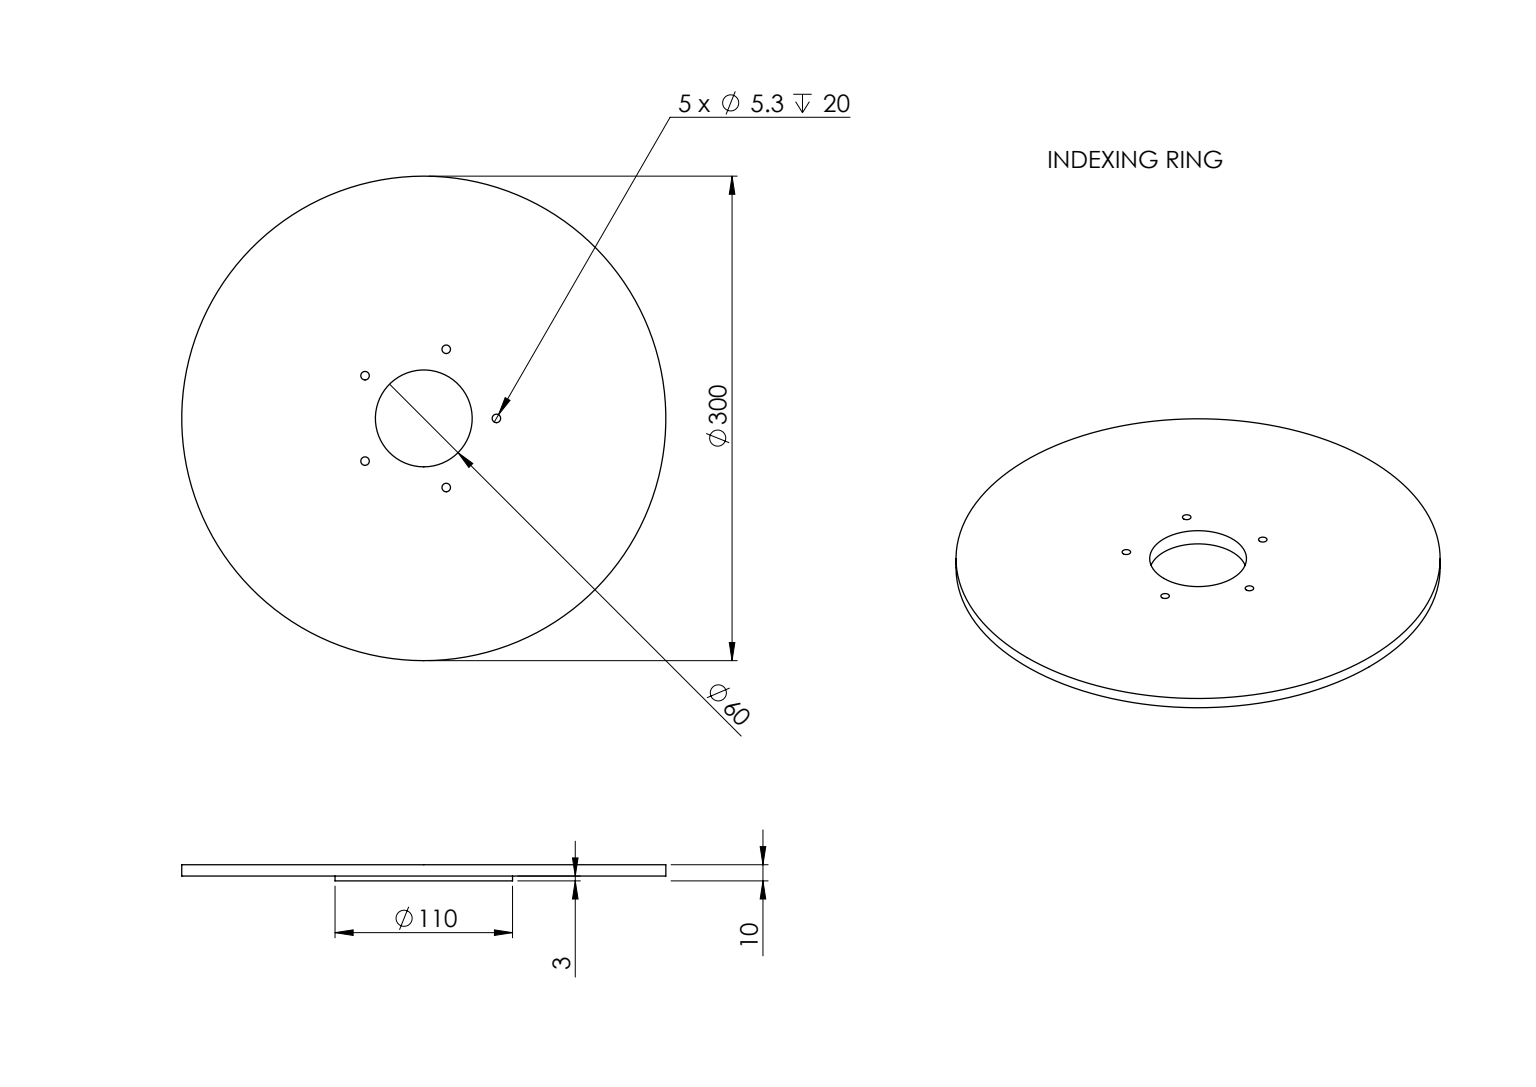
ISO-10303-21;
HEADER;
FILE_DESCRIPTION (('STEP AP214'),
    '1' );
FILE_NAME ('Indexing Ring.step',
    '2026-10-24T07:08:27',
    ( '' ),
    ( '' ),
    'SwSTEP 2.0',
    'SolidWorks 2026',
    '' );
FILE_SCHEMA (( 'AUTOMOTIVE_DESIGN' ));
ENDSEC;

DATA;
#5=CIRCLE ( 'NONE', #16107, 2.649999999999999467 ) ;
#16=ORIENTED_EDGE ( 'NONE', *, *, #15782, .F. ) ;
#43=AXIS2_PLACEMENT_3D ( 'NONE', #4578, #2974, #8946 ) ;
#70=DIRECTION ( 'NONE',  ( 0.000000000000000000, 0.000000000000000000, 1.000000000000000000 ) ) ;
#74=VECTOR ( 'NONE', #5888, 1000.000000000000000 ) ;
#109=DIRECTION ( 'NONE',  ( -0.000000000000000000, 1.000000000000000000, -0.000000000000000000 ) ) ;
#135=CARTESIAN_POINT ( 'NONE',  ( 13.90576474687299680, 0.000000000000000000, 42.79754323328179311 ) ) ;
#142=LINE ( 'NONE', #1937, #2927 ) ;
#166=CYLINDRICAL_SURFACE ( 'NONE', #15609, 30.00000000000000000 ) ;
#204=CYLINDRICAL_SURFACE ( 'NONE', #43, 55.00000000000000000 ) ;
#220=EDGE_CURVE ( 'NONE', #7351, #4921, #14999, .T. ) ;
#273=ORIENTED_EDGE ( 'NONE', *, *, #14374, .F. ) ;
#286=DIRECTION ( 'NONE',  ( -0.000000000000000000, -1.000000000000000000, -0.000000000000000000 ) ) ;
#301=ORIENTED_EDGE ( 'NONE', *, *, #12426, .F. ) ;
#305=EDGE_CURVE ( 'NONE', #13142, #9008, #11661, .T. ) ;
#340=ORIENTED_EDGE ( 'NONE', *, *, #305, .F. ) ;
#390=DIRECTION ( 'NONE',  ( 0.000000000000000000, -1.000000000000000000, 0.000000000000000000 ) ) ;
#402=EDGE_CURVE ( 'NONE', #11928, #9088, #2271, .T. ) ;
#413=CARTESIAN_POINT ( 'NONE',  ( 0.000000000000000000, 3.000000000000000000, 0.000000000000000000 ) ) ;
#469=DIRECTION ( 'NONE',  ( -0.000000000000000000, 1.000000000000000000, -0.000000000000000000 ) ) ;
#486=( LENGTH_UNIT ( ) NAMED_UNIT ( * ) SI_UNIT ( .MILLI., .METRE. ) );
#520=ORIENTED_EDGE ( 'NONE', *, *, #14011, .T. ) ;
#640=ORIENTED_EDGE ( 'NONE', *, *, #15047, .T. ) ;
#641=EDGE_CURVE ( 'NONE', #14362, #16890, #13288, .T. ) ;
#689=AXIS2_PLACEMENT_3D ( 'NONE', #18645, #7031, #2265 ) ;
#779=AXIS2_PLACEMENT_3D ( 'NONE', #6879, #12893, #15840 ) ;
#880=EDGE_CURVE ( 'NONE', #14362, #3677, #9321, .T. ) ;
#898=CARTESIAN_POINT ( 'NONE',  ( 13.90576474687263264, 0.000000000000000000, -42.79754323328189969 ) ) ;
#940=DIRECTION ( 'NONE',  ( 0.000000000000000000, 0.000000000000000000, 1.000000000000000000 ) ) ;
#955=ORIENTED_EDGE ( 'NONE', *, *, #4704, .T. ) ;
#967=CARTESIAN_POINT ( 'NONE',  ( 13.90576474687263264, 0.000000000000000000, -40.14754323328190111 ) ) ;
#970=ORIENTED_EDGE ( 'NONE', *, *, #12368, .T. ) ;
#982=CARTESIAN_POINT ( 'NONE',  ( 0.000000000000000000, 10.00000000000000000, -30.00000000000000000 ) ) ;
#991=DIRECTION ( 'NONE',  ( 0.000000000000000000, 0.000000000000000000, 1.000000000000000000 ) ) ;
#1029=EDGE_LOOP ( 'NONE', ( #970, #3446 ) ) ;
#1070=CARTESIAN_POINT ( 'NONE',  ( -36.40576474687271258, 10.00000000000000000, -26.45033635316118747 ) ) ;
#1105=AXIS2_PLACEMENT_3D ( 'NONE', #4053, #17378, #12810 ) ;
#1236=CYLINDRICAL_SURFACE ( 'NONE', #689, 2.649999999999999467 ) ;
#1286=AXIS2_PLACEMENT_3D ( 'NONE', #17811, #8951, #10577 ) ;
#1294=DIRECTION ( 'NONE',  ( 0.000000000000000000, 0.000000000000000000, 1.000000000000000000 ) ) ;
#1343=EDGE_LOOP ( 'NONE', ( #520, #9190 ) ) ;
#1397=EDGE_LOOP ( 'NONE', ( #11377, #14520, #10547, #14301 ) ) ;
#1452=CIRCLE ( 'NONE', #12089, 2.649999999999999467 ) ;
#1510=ADVANCED_FACE ( 'NONE', ( #15262, #2212 ), #17837, .T. ) ;
#1524=LINE ( 'NONE', #13055, #14054 ) ;
#1532=DIRECTION ( 'NONE',  ( 0.000000000000000000, -1.000000000000000000, 0.000000000000000000 ) ) ;
#1540=ORIENTED_EDGE ( 'NONE', *, *, #641, .F. ) ;
#1585=ORIENTED_EDGE ( 'NONE', *, *, #17375, .F. ) ;
#1675=AXIS2_PLACEMENT_3D ( 'NONE', #9927, #15556, #991 ) ;
#1709=AXIS2_PLACEMENT_3D ( 'NONE', #3286, #16430, #8983 ) ;
#1710=ADVANCED_FACE ( 'NONE', ( #9924 ), #17174, .F. ) ;
#1765=CARTESIAN_POINT ( 'NONE',  ( 0.000000000000000000, 3.000000000000000000, 0.000000000000000000 ) ) ;
#1859=DIRECTION ( 'NONE',  ( -0.000000000000000000, -1.000000000000000000, -0.000000000000000000 ) ) ;
#1868=LINE ( 'NONE', #16163, #9313 ) ;
#1911=DIRECTION ( 'NONE',  ( 1.000000000000000000, 0.000000000000000000, 0.000000000000000000 ) ) ;
#1926=ORIENTED_EDGE ( 'NONE', *, *, #12328, .F. ) ;
#1937=CARTESIAN_POINT ( 'NONE',  ( -36.40576474687271258, 10.00000000000000000, -29.10033635316118961 ) ) ;
#1938=LINE ( 'NONE', #6417, #10148 ) ;
#1963=CARTESIAN_POINT ( 'NONE',  ( -36.40576474687271258, 10.00000000000000000, -29.10033635316118961 ) ) ;
#1966=DIRECTION ( 'NONE',  ( -0.000000000000000000, 1.000000000000000000, -0.000000000000000000 ) ) ;
#1971=AXIS2_PLACEMENT_3D ( 'NONE', #11706, #4557, #7409 ) ;
#1981=CARTESIAN_POINT ( 'NONE',  ( 45.00000000000000000, 10.00000000000000000, -2.650000000000511946 ) ) ;
#1996=EDGE_LOOP ( 'NONE', ( #7930, #18641, #8266, #16907 ) ) ;
#2097=AXIS2_PLACEMENT_3D ( 'NONE', #16593, #15458, #3830 ) ;
#2107=VERTEX_POINT ( 'NONE', #967 ) ;
#2121=CYLINDRICAL_SURFACE ( 'NONE', #16679, 150.0000000000000284 ) ;
#2123=DIRECTION ( 'NONE',  ( 0.000000000000000000, -1.000000000000000000, 0.000000000000000000 ) ) ;
#2158=ORIENTED_EDGE ( 'NONE', *, *, #18549, .T. ) ;
#2212=FACE_OUTER_BOUND ( 'NONE', #3227, .T. ) ;
#2223=CLOSED_SHELL ( 'NONE', ( #15200, #17927, #1710, #5636, #4878, #2825, #17976, #16218, #14114, #15768, #13678, #3090, #12859, #4334, #4412, #8329, #14903, #1510, #9932 ) ) ;
#2253=CYLINDRICAL_SURFACE ( 'NONE', #7817, 2.649999999999999467 ) ;
#2265=DIRECTION ( 'NONE',  ( 0.000000000000000000, 0.000000000000000000, 1.000000000000000000 ) ) ;
#2271=LINE ( 'NONE', #15705, #10103 ) ;
#2500=DIRECTION ( 'NONE',  ( 0.000000000000000000, -1.000000000000000000, 0.000000000000000000 ) ) ;
#2501=DIRECTION ( 'NONE',  ( -0.000000000000000000, 1.000000000000000000, -0.000000000000000000 ) ) ;
#2534=DIRECTION ( 'NONE',  ( -0.000000000000000000, 1.000000000000000000, -0.000000000000000000 ) ) ;
#2568=DIRECTION ( 'NONE',  ( -0.000000000000000000, 1.000000000000000000, -0.000000000000000000 ) ) ;
#2580=EDGE_LOOP ( 'NONE', ( #4963, #18151 ) ) ;
#2605=ORIENTED_EDGE ( 'NONE', *, *, #12034, .T. ) ;
#2612=CIRCLE ( 'NONE', #6253, 2.649999999999999467 ) ;
#2736=FACE_BOUND ( 'NONE', #8126, .T. ) ;
#2771=ORIENTED_EDGE ( 'NONE', *, *, #13030, .F. ) ;
#2778=ORIENTED_EDGE ( 'NONE', *, *, #402, .T. ) ;
#2794=SURFACE_STYLE_USAGE ( .BOTH. , #11462 ) ;
#2801=CIRCLE ( 'NONE', #12208, 150.0000000000000000 ) ;
#2803=PLANE ( 'NONE',  #1105 ) ;
#2804=CARTESIAN_POINT ( 'NONE',  ( 45.00000000000000000, 10.00000000000000000, 2.649999999999487432 ) ) ;
#2825=ADVANCED_FACE ( 'NONE', ( #5792 ), #4360, .F. ) ;
#2829=ORIENTED_EDGE ( 'NONE', *, *, #16831, .T. ) ;
#2845=AXIS2_PLACEMENT_3D ( 'NONE', #15238, #14861, #10564 ) ;
#2891=EDGE_CURVE ( 'NONE', #3956, #15653, #1868, .T. ) ;
#2903=CARTESIAN_POINT ( 'NONE',  ( 6.735557395310442615E-15, 0.000000000000000000, 55.00000000000000000 ) ) ;
#2913=AXIS2_PLACEMENT_3D ( 'NONE', #6516, #7946, #6621 ) ;
#2927=VECTOR ( 'NONE', #13281, 1000.000000000000000 ) ;
#2974=DIRECTION ( 'NONE',  ( -0.000000000000000000, -1.000000000000000000, -0.000000000000000000 ) ) ;
#3025=ORIENTED_EDGE ( 'NONE', *, *, #8650, .T. ) ;
#3090=ADVANCED_FACE ( 'NONE', ( #5286 ), #12440, .F. ) ;
#3120=EDGE_CURVE ( 'NONE', #18403, #16590, #6572, .T. ) ;
#3227=EDGE_LOOP ( 'NONE', ( #14533, #10465 ) ) ;
#3286=CARTESIAN_POINT ( 'NONE',  ( -36.40576474687247099, 10.00000000000000000, 26.45033635316149301 ) ) ;
#3310=EDGE_CURVE ( 'NONE', #6304, #3994, #142, .T. ) ;
#3354=CARTESIAN_POINT ( 'NONE',  ( 45.00000000000000000, 0.000000000000000000, 2.649999999999487432 ) ) ;
#3396=CIRCLE ( 'NONE', #1286, 2.649999999999999467 ) ;
#3446=ORIENTED_EDGE ( 'NONE', *, *, #12426, .T. ) ;
#3501=CIRCLE ( 'NONE', #4120, 55.00000000000000000 ) ;
#3517=VERTEX_POINT ( 'NONE', #15824 ) ;
#3585=DIRECTION ( 'NONE',  ( 0.000000000000000000, 0.000000000000000000, -1.000000000000000000 ) ) ;
#3631=ORIENTED_EDGE ( 'NONE', *, *, #12034, .F. ) ;
#3632=CARTESIAN_POINT ( 'NONE',  ( 0.000000000000000000, 0.000000000000000000, 0.000000000000000000 ) ) ;
#3677=VERTEX_POINT ( 'NONE', #6089 ) ;
#3705=EDGE_LOOP ( 'NONE', ( #16152, #4220 ) ) ;
#3735=VECTOR ( 'NONE', #12593, 1000.000000000000000 ) ;
#3737=ORIENTED_EDGE ( 'NONE', *, *, #17718, .F. ) ;
#3785=EDGE_LOOP ( 'NONE', ( #10703, #14581, #9081, #11061 ) ) ;
#3830=DIRECTION ( 'NONE',  ( 0.000000000000000000, 0.000000000000000000, -1.000000000000000000 ) ) ;
#3940=DIRECTION ( 'NONE',  ( 0.000000000000000000, 1.000000000000000000, 0.000000000000000000 ) ) ;
#3956=VERTEX_POINT ( 'NONE', #7399 ) ;
#3994=VERTEX_POINT ( 'NONE', #1963 ) ;
#4039=DIRECTION ( 'NONE',  ( 0.000000000000000000, 0.000000000000000000, 1.000000000000000000 ) ) ;
#4045=CARTESIAN_POINT ( 'NONE',  ( 45.00000000000000000, 0.000000000000000000, -5.120903701083534543E-13 ) ) ;
#4053=CARTESIAN_POINT ( 'NONE',  ( 0.000000000000000000, 0.000000000000000000, 0.000000000000000000 ) ) ;
#4120=AXIS2_PLACEMENT_3D ( 'NONE', #18310, #11060, #16887 ) ;
#4185=EDGE_CURVE ( 'NONE', #9008, #13142, #2612, .T. ) ;
#4198=CARTESIAN_POINT ( 'NONE',  ( -36.40576474687247099, 10.00000000000000000, 29.10033635316149514 ) ) ;
#4206=FACE_OUTER_BOUND ( 'NONE', #12915, .T. ) ;
#4220=ORIENTED_EDGE ( 'NONE', *, *, #17207, .T. ) ;
#4246=DIRECTION ( 'NONE',  ( 0.000000000000000000, 1.000000000000000000, 0.000000000000000000 ) ) ;
#4296=ORIENTED_EDGE ( 'NONE', *, *, #9114, .T. ) ;
#4313=CIRCLE ( 'NONE', #6737, 150.0000000000000284 ) ;
#4334=ADVANCED_FACE ( 'NONE', ( #10146 ), #17204, .F. ) ;
#4355=FACE_OUTER_BOUND ( 'NONE', #10583, .T. ) ;
#4360=CYLINDRICAL_SURFACE ( 'NONE', #12135, 2.649999999999999467 ) ;
#4363=VERTEX_POINT ( 'NONE', #5495 ) ;
#4412=ADVANCED_FACE ( 'NONE', ( #13572 ), #7653, .F. ) ;
#4424=VECTOR ( 'NONE', #9470, 1000.000000000000000 ) ;
#4439=DIRECTION ( 'NONE',  ( -0.000000000000000000, 1.000000000000000000, -0.000000000000000000 ) ) ;
#4464=FACE_OUTER_BOUND ( 'NONE', #5126, .T. ) ;
#4465=AXIS2_PLACEMENT_3D ( 'NONE', #5371, #9941, #15755 ) ;
#4479=CARTESIAN_POINT ( 'NONE',  ( -36.40576474687271258, 10.00000000000000000, -26.45033635316118747 ) ) ;
#4491=( LENGTH_UNIT ( ) NAMED_UNIT ( * ) SI_UNIT ( .MILLI., .METRE. ) );
#4504=( NAMED_UNIT ( * ) PLANE_ANGLE_UNIT ( ) SI_UNIT ( $, .RADIAN. ) );
#4530=ORIENTED_EDGE ( 'NONE', *, *, #17601, .F. ) ;
#4557=DIRECTION ( 'NONE',  ( -0.000000000000000000, -1.000000000000000000, -0.000000000000000000 ) ) ;
#4578=CARTESIAN_POINT ( 'NONE',  ( 0.000000000000000000, 3.000000000000000000, 0.000000000000000000 ) ) ;
#4581=( NAMED_UNIT ( * ) PLANE_ANGLE_UNIT ( ) SI_UNIT ( $, .RADIAN. ) );
#4630=APPLICATION_CONTEXT ( 'automotive_design' ) ;
#4662=CYLINDRICAL_SURFACE ( 'NONE', #14552, 2.649999999999999467 ) ;
#4673=PRODUCT_DEFINITION ( 'UNKNOWN', '', #8673, #14538 ) ;
#4704=EDGE_CURVE ( 'NONE', #16890, #11456, #12037, .T. ) ;
#4754=FACE_OUTER_BOUND ( 'NONE', #5207, .T. ) ;
#4769=AXIS2_PLACEMENT_3D ( 'NONE', #17245, #16087, #10275 ) ;
#4796=DIRECTION ( 'NONE',  ( -0.000000000000000000, 1.000000000000000000, -0.000000000000000000 ) ) ;
#4878=ADVANCED_FACE ( 'NONE', ( #4464 ), #9998, .F. ) ;
#4911=EDGE_CURVE ( 'NONE', #16590, #14829, #7043, .T. ) ;
#4921=VERTEX_POINT ( 'NONE', #18756 ) ;
#4963=ORIENTED_EDGE ( 'NONE', *, *, #9468, .T. ) ;
#4969=COLOUR_RGB ( '',0.8941176470588234615, 0.8941176470588234615, 0.8941176470588234615 ) ;
#5121=ORIENTED_EDGE ( 'NONE', *, *, #17375, .T. ) ;
#5126=EDGE_LOOP ( 'NONE', ( #10625, #10506, #16849, #1585 ) ) ;
#5157=EDGE_CURVE ( 'NONE', #9088, #10404, #9039, .T. ) ;
#5177=ORIENTED_EDGE ( 'NONE', *, *, #17207, .F. ) ;
#5195=DIRECTION ( 'NONE',  ( -0.000000000000000000, -1.000000000000000000, -0.000000000000000000 ) ) ;
#5201=DIRECTION ( 'NONE',  ( -0.000000000000000000, 1.000000000000000000, -0.000000000000000000 ) ) ;
#5207=EDGE_LOOP ( 'NONE', ( #10879, #7424, #17278, #10605 ) ) ;
#5276=CARTESIAN_POINT ( 'NONE',  ( 13.90576474687299680, 10.00000000000000000, 40.14754323328178742 ) ) ;
#5286=FACE_OUTER_BOUND ( 'NONE', #18515, .T. ) ;
#5365=CIRCLE ( 'NONE', #16947, 2.649999999999999467 ) ;
#5371=CARTESIAN_POINT ( 'NONE',  ( 0.000000000000000000, 10.00000000000000000, 0.000000000000000000 ) ) ;
#5393=DIRECTION ( 'NONE',  ( 0.000000000000000000, 0.000000000000000000, 1.000000000000000000 ) ) ;
#5472=AXIS2_PLACEMENT_3D ( 'NONE', #13696, #1966, #18155 ) ;
#5485=DIRECTION ( 'NONE',  ( 0.000000000000000000, -1.000000000000000000, 0.000000000000000000 ) ) ;
#5494=ORIENTED_EDGE ( 'NONE', *, *, #7706, .T. ) ;
#5495=CARTESIAN_POINT ( 'NONE',  ( 45.00000000000000000, 0.000000000000000000, -2.650000000000511946 ) ) ;
#5555=CARTESIAN_POINT ( 'NONE',  ( -36.40576474687271258, 10.00000000000000000, -26.45033635316118747 ) ) ;
#5563=DIRECTION ( 'NONE',  ( 0.000000000000000000, 0.000000000000000000, 1.000000000000000000 ) ) ;
#5578=DIRECTION ( 'NONE',  ( 0.000000000000000000, 1.000000000000000000, 0.000000000000000000 ) ) ;
#5593=EDGE_LOOP ( 'NONE', ( #5669, #6351, #10190, #1540 ) ) ;
#5636=ADVANCED_FACE ( 'NONE', ( #4355 ), #8821, .F. ) ;
#5649=SURFACE_STYLE_FILL_AREA ( #15844 ) ;
#5650=DIRECTION ( 'NONE',  ( 0.000000000000000000, 0.000000000000000000, 1.000000000000000000 ) ) ;
#5659=FACE_BOUND ( 'NONE', #2580, .T. ) ;
#5668=VECTOR ( 'NONE', #286, 1000.000000000000000 ) ;
#5669=ORIENTED_EDGE ( 'NONE', *, *, #880, .T. ) ;
#5682=AXIS2_PLACEMENT_3D ( 'NONE', #1070, #15736, #8401 ) ;
#5700=ORIENTED_EDGE ( 'NONE', *, *, #8890, .F. ) ;
#5706=EDGE_LOOP ( 'NONE', ( #8634, #340 ) ) ;
#5712=ORIENTED_EDGE ( 'NONE', *, *, #3120, .F. ) ;
#5786=EDGE_LOOP ( 'NONE', ( #9980, #17221 ) ) ;
#5792=FACE_OUTER_BOUND ( 'NONE', #18175, .T. ) ;
#5804=FACE_OUTER_BOUND ( 'NONE', #17196, .T. ) ;
#5850=CARTESIAN_POINT ( 'NONE',  ( -36.40576474687247099, 0.000000000000000000, 23.80033635316149443 ) ) ;
#5888=DIRECTION ( 'NONE',  ( -0.000000000000000000, 1.000000000000000000, -0.000000000000000000 ) ) ;
#5929=DIRECTION ( 'NONE',  ( 0.000000000000000000, 1.000000000000000000, 0.000000000000000000 ) ) ;
#5946=LINE ( 'NONE', #8449, #15377 ) ;
#6047=DIRECTION ( 'NONE',  ( -0.000000000000000000, -1.000000000000000000, -0.000000000000000000 ) ) ;
#6089=CARTESIAN_POINT ( 'NONE',  ( 3.673940397442059178E-15, 10.00000000000000000, 30.00000000000000000 ) ) ;
#6119=EDGE_CURVE ( 'NONE', #18371, #8784, #14558, .T. ) ;
#6123=CARTESIAN_POINT ( 'NONE',  ( -36.40576474687271258, 10.00000000000000000, -23.80033635316118890 ) ) ;
#6236=CARTESIAN_POINT ( 'NONE',  ( 6.735557395310442615E-15, 3.000000000000000000, 55.00000000000000000 ) ) ;
#6253=AXIS2_PLACEMENT_3D ( 'NONE', #9396, #5201, #5393 ) ;
#6254=CIRCLE ( 'NONE', #18107, 2.649999999999999467 ) ;
#6261=CARTESIAN_POINT ( 'NONE',  ( 0.000000000000000000, 3.000000000000000000, 0.000000000000000000 ) ) ;
#6304=VERTEX_POINT ( 'NONE', #15354 ) ;
#6337=PRODUCT ( 'Indexing Ring', 'Indexing Ring', '', ( #10128 ) ) ;
#6351=ORIENTED_EDGE ( 'NONE', *, *, #17601, .T. ) ;
#6361=STYLED_ITEM('',(#18890),#15935);
#6375=DIRECTION ( 'NONE',  ( 0.000000000000000000, 0.000000000000000000, 1.000000000000000000 ) ) ;
#6396=( NAMED_UNIT ( * ) SI_UNIT ( $, .STERADIAN. ) SOLID_ANGLE_UNIT ( ) );
#6417=CARTESIAN_POINT ( 'NONE',  ( 13.90576474687263264, 10.00000000000000000, -45.44754323328189827 ) ) ;
#6516=CARTESIAN_POINT ( 'NONE',  ( 0.000000000000000000, 10.00000000000000000, 0.000000000000000000 ) ) ;
#6540=CIRCLE ( 'NONE', #779, 2.649999999999999467 ) ;
#6572=CIRCLE ( 'NONE', #8994, 2.649999999999999467 ) ;
#6618=VECTOR ( 'NONE', #14346, 1000.000000000000000 ) ;
#6621=DIRECTION ( 'NONE',  ( 0.000000000000000000, 0.000000000000000000, 1.000000000000000000 ) ) ;
#6630=AXIS2_PLACEMENT_3D ( 'NONE', #7074, #10212, #5563 ) ;
#6668=MECHANICAL_DESIGN_GEOMETRIC_PRESENTATION_REPRESENTATION('',(#6361),#15787);
#6701=CARTESIAN_POINT ( 'NONE',  ( 0.000000000000000000, 0.000000000000000000, -30.00000000000000000 ) ) ;
#6713=ORIENTED_EDGE ( 'NONE', *, *, #220, .F. ) ;
#6719=CARTESIAN_POINT ( 'NONE',  ( 0.000000000000000000, 0.000000000000000000, 0.000000000000000000 ) ) ;
#6724=DIRECTION ( 'NONE',  ( 0.000000000000000000, 0.000000000000000000, -1.000000000000000000 ) ) ;
#6737=AXIS2_PLACEMENT_3D ( 'NONE', #17449, #8504, #12100 ) ;
#6755=AXIS2_PLACEMENT_3D ( 'NONE', #11426, #11336, #17154 ) ;
#6777=AXIS2_PLACEMENT_3D ( 'NONE', #14577, #1532, #7334 ) ;
#6822=CARTESIAN_POINT ( 'NONE',  ( 13.90576474687263264, 10.00000000000000000, -42.79754323328189969 ) ) ;
#6833=ORIENTED_EDGE ( 'NONE', *, *, #3120, .T. ) ;
#6849=DIRECTION ( 'NONE',  ( 0.000000000000000000, 0.000000000000000000, 1.000000000000000000 ) ) ;
#6856=CARTESIAN_POINT ( 'NONE',  ( 45.00000000000000000, 10.00000000000000000, -5.120903701083534543E-13 ) ) ;
#6879=CARTESIAN_POINT ( 'NONE',  ( -36.40576474687271258, 0.000000000000000000, -26.45033635316118747 ) ) ;
#6976=ORIENTED_EDGE ( 'NONE', *, *, #7706, .F. ) ;
#7000=FACE_BOUND ( 'NONE', #11546, .T. ) ;
#7031=DIRECTION ( 'NONE',  ( -0.000000000000000000, 1.000000000000000000, -0.000000000000000000 ) ) ;
#7043=LINE ( 'NONE', #4198, #17854 ) ;
#7047=CIRCLE ( 'NONE', #17651, 2.649999999999999467 ) ;
#7059=ORIENTED_EDGE ( 'NONE', *, *, #14529, .F. ) ;
#7061=CIRCLE ( 'NONE', #6755, 2.649999999999999467 ) ;
#7074=CARTESIAN_POINT ( 'NONE',  ( -36.40576474687247099, 10.00000000000000000, 26.45033635316149301 ) ) ;
#7107=CARTESIAN_POINT ( 'NONE',  ( 0.000000000000000000, 3.000000000000000000, -55.00000000000000000 ) ) ;
#7198=CARTESIAN_POINT ( 'NONE',  ( 13.90576474687263264, 10.00000000000000000, -40.14754323328190111 ) ) ;
#7208=DIRECTION ( 'NONE',  ( 0.000000000000000000, 0.000000000000000000, -1.000000000000000000 ) ) ;
#7315=CARTESIAN_POINT ( 'NONE',  ( 13.90576474687299680, 0.000000000000000000, 45.44754323328179169 ) ) ;
#7317=CARTESIAN_POINT ( 'NONE',  ( 13.90576474687299680, 10.00000000000000000, 45.44754323328179169 ) ) ;
#7322=DIRECTION ( 'NONE',  ( 1.000000000000000000, 0.000000000000000000, 0.000000000000000000 ) ) ;
#7334=DIRECTION ( 'NONE',  ( 0.000000000000000000, 0.000000000000000000, -1.000000000000000000 ) ) ;
#7351=VERTEX_POINT ( 'NONE', #2903 ) ;
#7399=CARTESIAN_POINT ( 'NONE',  ( -36.40576474687271258, 0.000000000000000000, -23.80033635316118890 ) ) ;
#7409=DIRECTION ( 'NONE',  ( 0.000000000000000000, 0.000000000000000000, -1.000000000000000000 ) ) ;
#7424=ORIENTED_EDGE ( 'NONE', *, *, #12368, .F. ) ;
#7426=FACE_OUTER_BOUND ( 'NONE', #14178, .T. ) ;
#7519=DIRECTION ( 'NONE',  ( 0.000000000000000000, 0.000000000000000000, 1.000000000000000000 ) ) ;
#7562=AXIS2_PLACEMENT_3D ( 'NONE', #13153, #109, #7519 ) ;
#7627=CARTESIAN_POINT ( 'NONE',  ( 13.90576474687263264, 10.00000000000000000, -45.44754323328189827 ) ) ;
#7653=CYLINDRICAL_SURFACE ( 'NONE', #1709, 2.649999999999999467 ) ;
#7706=EDGE_CURVE ( 'NONE', #14393, #14829, #15759, .T. ) ;
#7713=VERTEX_POINT ( 'NONE', #18605 ) ;
#7718=EDGE_CURVE ( 'NONE', #17227, #4363, #1452, .T. ) ;
#7734=EDGE_LOOP ( 'NONE', ( #11489, #16 ) ) ;
#7817=AXIS2_PLACEMENT_3D ( 'NONE', #6822, #8062, #940 ) ;
#7930=ORIENTED_EDGE ( 'NONE', *, *, #18573, .F. ) ;
#7946=DIRECTION ( 'NONE',  ( 0.000000000000000000, 1.000000000000000000, 0.000000000000000000 ) ) ;
#8017=AXIS2_PLACEMENT_3D ( 'NONE', #12801, #14324, #9934 ) ;
#8062=DIRECTION ( 'NONE',  ( -0.000000000000000000, 1.000000000000000000, -0.000000000000000000 ) ) ;
#8100=CARTESIAN_POINT ( 'NONE',  ( 3.673940397442059178E-15, 0.000000000000000000, 30.00000000000000000 ) ) ;
#8126=EDGE_LOOP ( 'NONE', ( #11049, #1926 ) ) ;
#8157=AXIS2_PLACEMENT_3D ( 'NONE', #6719, #5485, #12613 ) ;
#8206=CYLINDRICAL_SURFACE ( 'NONE', #14182, 2.649999999999999467 ) ;
#8244=DIRECTION ( 'NONE',  ( 0.000000000000000000, 0.000000000000000000, 1.000000000000000000 ) ) ;
#8255=EDGE_LOOP ( 'NONE', ( #640, #6833 ) ) ;
#8266=ORIENTED_EDGE ( 'NONE', *, *, #15061, .T. ) ;
#8292=AXIS2_PLACEMENT_3D ( 'NONE', #15139, #16469, #6375 ) ;
#8329=ADVANCED_FACE ( 'NONE', ( #4754 ), #4662, .F. ) ;
#8337=DIRECTION ( 'NONE',  ( -0.000000000000000000, 1.000000000000000000, -0.000000000000000000 ) ) ;
#8357=CARTESIAN_POINT ( 'NONE',  ( -36.40576474687247099, 0.000000000000000000, 29.10033635316149514 ) ) ;
#8374=VECTOR ( 'NONE', #8633, 1000.000000000000000 ) ;
#8401=DIRECTION ( 'NONE',  ( 0.000000000000000000, 0.000000000000000000, 1.000000000000000000 ) ) ;
#8434=EDGE_CURVE ( 'NONE', #15653, #3994, #15784, .T. ) ;
#8449=CARTESIAN_POINT ( 'NONE',  ( 6.735557395310442615E-15, 3.000000000000000000, 55.00000000000000000 ) ) ;
#8504=DIRECTION ( 'NONE',  ( 0.000000000000000000, 1.000000000000000000, 0.000000000000000000 ) ) ;
#8521=DIRECTION ( 'NONE',  ( 0.000000000000000000, 1.000000000000000000, 0.000000000000000000 ) ) ;
#8531=CARTESIAN_POINT ( 'NONE',  ( 13.90576474687299680, 10.00000000000000000, 42.79754323328179311 ) ) ;
#8553=ORIENTED_EDGE ( 'NONE', *, *, #17106, .F. ) ;
#8558=DIRECTION ( 'NONE',  ( 0.000000000000000000, 0.000000000000000000, 1.000000000000000000 ) ) ;
#8596=PRESENTATION_STYLE_ASSIGNMENT (( #2794 ) ) ;
#8633=DIRECTION ( 'NONE',  ( -0.000000000000000000, -1.000000000000000000, -0.000000000000000000 ) ) ;
#8634=ORIENTED_EDGE ( 'NONE', *, *, #4185, .F. ) ;
#8650=EDGE_CURVE ( 'NONE', #11456, #16890, #18530, .T. ) ;
#8673=PRODUCT_DEFINITION_FORMATION_WITH_SPECIFIED_SOURCE ( 'ANY', '', #6337, .NOT_KNOWN. ) ;
#8676=AXIS2_PLACEMENT_3D ( 'NONE', #8814, #13114, #10149 ) ;
#8724=AXIS2_PLACEMENT_3D ( 'NONE', #6261, #2500, #7322 ) ;
#8729=DIRECTION ( 'NONE',  ( 0.000000000000000000, 0.000000000000000000, 1.000000000000000000 ) ) ;
#8784=VERTEX_POINT ( 'NONE', #7315 ) ;
#8814=CARTESIAN_POINT ( 'NONE',  ( 0.000000000000000000, 10.00000000000000000, 0.000000000000000000 ) ) ;
#8821=CYLINDRICAL_SURFACE ( 'NONE', #15147, 2.649999999999999467 ) ;
#8890=EDGE_CURVE ( 'NONE', #7713, #10053, #12464, .T. ) ;
#8946=DIRECTION ( 'NONE',  ( 0.000000000000000000, 0.000000000000000000, -1.000000000000000000 ) ) ;
#8951=DIRECTION ( 'NONE',  ( 0.000000000000000000, 1.000000000000000000, 0.000000000000000000 ) ) ;
#8983=DIRECTION ( 'NONE',  ( 0.000000000000000000, 0.000000000000000000, 1.000000000000000000 ) ) ;
#8994=AXIS2_PLACEMENT_3D ( 'NONE', #11666, #5578, #13105 ) ;
#9008=VERTEX_POINT ( 'NONE', #17973 ) ;
#9021=ORIENTED_EDGE ( 'NONE', *, *, #17230, .F. ) ;
#9039=CIRCLE ( 'NONE', #8724, 150.0000000000000000 ) ;
#9064=EDGE_CURVE ( 'NONE', #3517, #17226, #5, .T. ) ;
#9069=CIRCLE ( 'NONE', #2097, 55.00000000000000000 ) ;
#9081=ORIENTED_EDGE ( 'NONE', *, *, #4911, .T. ) ;
#9088=VERTEX_POINT ( 'NONE', #11296 ) ;
#9114=EDGE_CURVE ( 'NONE', #4363, #13142, #17030, .T. ) ;
#9148=CARTESIAN_POINT ( 'NONE',  ( 13.90576474687263264, 0.000000000000000000, -45.44754323328189827 ) ) ;
#9190=ORIENTED_EDGE ( 'NONE', *, *, #17106, .T. ) ;
#9212=ORIENTED_EDGE ( 'NONE', *, *, #7718, .F. ) ;
#9313=VECTOR ( 'NONE', #17966, 1000.000000000000000 ) ;
#9321=CIRCLE ( 'NONE', #4465, 30.00000000000000000 ) ;
#9369=EDGE_CURVE ( 'NONE', #17227, #9008, #10045, .T. ) ;
#9380=AXIS2_PLACEMENT_3D ( 'NONE', #11376, #8521, #1294 ) ;
#9396=CARTESIAN_POINT ( 'NONE',  ( 45.00000000000000000, 10.00000000000000000, -5.120903701083534543E-13 ) ) ;
#9468=EDGE_CURVE ( 'NONE', #2107, #17109, #9742, .T. ) ;
#9470=DIRECTION ( 'NONE',  ( -0.000000000000000000, 1.000000000000000000, -0.000000000000000000 ) ) ;
#9506=ORIENTED_EDGE ( 'NONE', *, *, #4911, .F. ) ;
#9542=CARTESIAN_POINT ( 'NONE',  ( -36.40576474687247099, 10.00000000000000000, 23.80033635316149443 ) ) ;
#9634=EDGE_LOOP ( 'NONE', ( #14943, #16876 ) ) ;
#9742=CIRCLE ( 'NONE', #12783, 2.649999999999999467 ) ;
#9780=CARTESIAN_POINT ( 'NONE',  ( -36.40576474687247099, 10.00000000000000000, 29.10033635316149514 ) ) ;
#9806=DIRECTION ( 'NONE',  ( 0.000000000000000000, 1.000000000000000000, 0.000000000000000000 ) ) ;
#9867=CARTESIAN_POINT ( 'NONE',  ( 13.90576474687263264, 10.00000000000000000, -42.79754323328189969 ) ) ;
#9881=EDGE_LOOP ( 'NONE', ( #13812, #18720, #18643, #3631 ) ) ;
#9893=CIRCLE ( 'NONE', #1675, 30.00000000000000000 ) ;
#9924=FACE_OUTER_BOUND ( 'NONE', #17870, .T. ) ;
#9927=CARTESIAN_POINT ( 'NONE',  ( 0.000000000000000000, 10.00000000000000000, 0.000000000000000000 ) ) ;
#9932=ADVANCED_FACE ( 'NONE', ( #7426 ), #204, .T. ) ;
#9934=DIRECTION ( 'NONE',  ( 1.000000000000000000, 0.000000000000000000, 0.000000000000000000 ) ) ;
#9941=DIRECTION ( 'NONE',  ( 0.000000000000000000, 1.000000000000000000, 0.000000000000000000 ) ) ;
#9967=FACE_OUTER_BOUND ( 'NONE', #1343, .T. ) ;
#9980=ORIENTED_EDGE ( 'NONE', *, *, #9064, .F. ) ;
#9998=CYLINDRICAL_SURFACE ( 'NONE', #4769, 2.649999999999999467 ) ;
#10006=DIRECTION ( 'NONE',  ( 0.000000000000000000, 0.000000000000000000, 1.000000000000000000 ) ) ;
#10045=LINE ( 'NONE', #2804, #18559 ) ;
#10053=VERTEX_POINT ( 'NONE', #10467 ) ;
#10103=VECTOR ( 'NONE', #16854, 1000.000000000000000 ) ;
#10128=PRODUCT_CONTEXT ( 'NONE', #4630, 'mechanical' ) ;
#10146=FACE_OUTER_BOUND ( 'NONE', #14633, .T. ) ;
#10148=VECTOR ( 'NONE', #4796, 1000.000000000000000 ) ;
#10149=DIRECTION ( 'NONE',  ( 0.000000000000000000, -0.000000000000000000, 1.000000000000000000 ) ) ;
#10161=STYLED_ITEM ( 'NONE', ( #8596 ), #13098 ) ;
#10190=ORIENTED_EDGE ( 'NONE', *, *, #4704, .F. ) ;
#10212=DIRECTION ( 'NONE',  ( -0.000000000000000000, 1.000000000000000000, -0.000000000000000000 ) ) ;
#10275=DIRECTION ( 'NONE',  ( 0.000000000000000000, 0.000000000000000000, 1.000000000000000000 ) ) ;
#10276=CYLINDRICAL_SURFACE ( 'NONE', #1971, 150.0000000000000284 ) ;
#10314=( NAMED_UNIT ( * ) SI_UNIT ( $, .STERADIAN. ) SOLID_ANGLE_UNIT ( ) );
#10326=CARTESIAN_POINT ( 'NONE',  ( 0.000000000000000000, 3.000000000000000000, -55.00000000000000000 ) ) ;
#10404=VERTEX_POINT ( 'NONE', #13850 ) ;
#10465=ORIENTED_EDGE ( 'NONE', *, *, #5157, .T. ) ;
#10467=CARTESIAN_POINT ( 'NONE',  ( 13.90576474687299680, 10.00000000000000000, 45.44754323328179169 ) ) ;
#10506=ORIENTED_EDGE ( 'NONE', *, *, #13877, .T. ) ;
#10522=CIRCLE ( 'NONE', #2913, 150.0000000000000284 ) ;
#10547=ORIENTED_EDGE ( 'NONE', *, *, #13030, .T. ) ;
#10564=DIRECTION ( 'NONE',  ( 0.000000000000000000, 0.000000000000000000, 1.000000000000000000 ) ) ;
#10573=EDGE_LOOP ( 'NONE', ( #16613, #7059 ) ) ;
#10577=DIRECTION ( 'NONE',  ( 0.000000000000000000, 0.000000000000000000, 1.000000000000000000 ) ) ;
#10583=EDGE_LOOP ( 'NONE', ( #5712, #2829, #5494, #9506 ) ) ;
#10605=ORIENTED_EDGE ( 'NONE', *, *, #8434, .T. ) ;
#10625=ORIENTED_EDGE ( 'NONE', *, *, #6119, .F. ) ;
#10703=ORIENTED_EDGE ( 'NONE', *, *, #16831, .F. ) ;
#10751=EDGE_CURVE ( 'NONE', #8784, #18371, #7047, .T. ) ;
#10765=VERTEX_POINT ( 'NONE', #10326 ) ;
#10879=ORIENTED_EDGE ( 'NONE', *, *, #3310, .F. ) ;
#10892=EDGE_LOOP ( 'NONE', ( #273, #16760, #2158, #15419 ) ) ;
#10970=LINE ( 'NONE', #9542, #3735 ) ;
#11049=ORIENTED_EDGE ( 'NONE', *, *, #880, .F. ) ;
#11058=DIRECTION ( 'NONE',  ( 0.000000000000000000, 0.000000000000000000, 1.000000000000000000 ) ) ;
#11060=DIRECTION ( 'NONE',  ( 0.000000000000000000, -1.000000000000000000, 0.000000000000000000 ) ) ;
#11061=ORIENTED_EDGE ( 'NONE', *, *, #17486, .T. ) ;
#11122=DIRECTION ( 'NONE',  ( 0.000000000000000000, 1.000000000000000000, 0.000000000000000000 ) ) ;
#11183=LINE ( 'NONE', #5276, #4424 ) ;
#11184=CARTESIAN_POINT ( 'NONE',  ( 13.90576474687263264, 0.000000000000000000, -42.79754323328189969 ) ) ;
#11231=CARTESIAN_POINT ( 'NONE',  ( 0.000000000000000000, 0.000000000000000000, 0.000000000000000000 ) ) ;
#11296=CARTESIAN_POINT ( 'NONE',  ( 1.836970198721029747E-14, 3.000000000000000000, 150.0000000000000000 ) ) ;
#11336=DIRECTION ( 'NONE',  ( -0.000000000000000000, 1.000000000000000000, -0.000000000000000000 ) ) ;
#11364=DIRECTION ( 'NONE',  ( 0.000000000000000000, 1.000000000000000000, 0.000000000000000000 ) ) ;
#11371=MECHANICAL_DESIGN_GEOMETRIC_PRESENTATION_REPRESENTATION('',(#10161),#15028);
#11376=CARTESIAN_POINT ( 'NONE',  ( 13.90576474687299680, 0.000000000000000000, 42.79754323328179311 ) ) ;
#11377=ORIENTED_EDGE ( 'NONE', *, *, #402, .F. ) ;
#11390=FACE_BOUND ( 'NONE', #5786, .T. ) ;
#11426=CARTESIAN_POINT ( 'NONE',  ( -36.40576474687247099, 10.00000000000000000, 26.45033635316149301 ) ) ;
#11456=VERTEX_POINT ( 'NONE', #8100 ) ;
#11462=SURFACE_SIDE_STYLE ('',( #5649 ) ) ;
#11475=FACE_OUTER_BOUND ( 'NONE', #9634, .T. ) ;
#11489=ORIENTED_EDGE ( 'NONE', *, *, #12257, .F. ) ;
#11511=FACE_OUTER_BOUND ( 'NONE', #5593, .T. ) ;
#11546=EDGE_LOOP ( 'NONE', ( #955, #3025 ) ) ;
#11562=( LENGTH_UNIT ( ) NAMED_UNIT ( * ) SI_UNIT ( .MILLI., .METRE. ) );
#11573=FACE_BOUND ( 'NONE', #8255, .T. ) ;
#11661=CIRCLE ( 'NONE', #2845, 2.649999999999999467 ) ;
#11666=CARTESIAN_POINT ( 'NONE',  ( -36.40576474687247099, 0.000000000000000000, 26.45033635316149301 ) ) ;
#11706=CARTESIAN_POINT ( 'NONE',  ( 0.000000000000000000, 10.00000000000000000, 0.000000000000000000 ) ) ;
#11751=DIRECTION ( 'NONE',  ( 0.000000000000000000, 0.000000000000000000, 1.000000000000000000 ) ) ;
#11755=CIRCLE ( 'NONE', #5682, 2.649999999999999467 ) ;
#11784=CARTESIAN_POINT ( 'NONE',  ( 0.000000000000000000, 10.00000000000000000, 0.000000000000000000 ) ) ;
#11873=DIRECTION ( 'NONE',  ( -0.000000000000000000, -1.000000000000000000, -0.000000000000000000 ) ) ;
#11928=VERTEX_POINT ( 'NONE', #12843 ) ;
#11943=ORIENTED_EDGE ( 'NONE', *, *, #641, .T. ) ;
#11967=ORIENTED_EDGE ( 'NONE', *, *, #13664, .F. ) ;
#12022=LINE ( 'NONE', #7107, #8374 ) ;
#12034=EDGE_CURVE ( 'NONE', #10765, #4921, #12022, .T. ) ;
#12037=CIRCLE ( 'NONE', #13269, 30.00000000000000000 ) ;
#12089=AXIS2_PLACEMENT_3D ( 'NONE', #4045, #11364, #5650 ) ;
#12100=DIRECTION ( 'NONE',  ( 0.000000000000000000, 0.000000000000000000, 1.000000000000000000 ) ) ;
#12133=ORIENTED_EDGE ( 'NONE', *, *, #17486, .F. ) ;
#12135=AXIS2_PLACEMENT_3D ( 'NONE', #15968, #14360, #8729 ) ;
#12208=AXIS2_PLACEMENT_3D ( 'NONE', #13449, #390, #1911 ) ;
#12257=EDGE_CURVE ( 'NONE', #10765, #15213, #3501, .T. ) ;
#12266=AXIS2_PLACEMENT_3D ( 'NONE', #17944, #13282, #17846 ) ;
#12328=EDGE_CURVE ( 'NONE', #3677, #14362, #9893, .T. ) ;
#12368=EDGE_CURVE ( 'NONE', #3956, #6304, #6540, .T. ) ;
#12426=EDGE_CURVE ( 'NONE', #6304, #3956, #6254, .T. ) ;
#12440=CYLINDRICAL_SURFACE ( 'NONE', #13278, 30.00000000000000000 ) ;
#12464=CIRCLE ( 'NONE', #5472, 2.649999999999999467 ) ;
#12491=ORIENTED_EDGE ( 'NONE', *, *, #10751, .T. ) ;
#12539=VECTOR ( 'NONE', #6047, 1000.000000000000000 ) ;
#12593=DIRECTION ( 'NONE',  ( -0.000000000000000000, 1.000000000000000000, -0.000000000000000000 ) ) ;
#12594=DIRECTION ( 'NONE',  ( 0.000000000000000000, 1.000000000000000000, 0.000000000000000000 ) ) ;
#12613=DIRECTION ( 'NONE',  ( 0.000000000000000000, 0.000000000000000000, -1.000000000000000000 ) ) ;
#12617=UNCERTAINTY_MEASURE_WITH_UNIT (LENGTH_MEASURE( 1.000000000000000082E-05 ), #4491, 'distance_accuracy_value', 'NONE');
#12692=CARTESIAN_POINT ( 'NONE',  ( 0.000000000000000000, 10.00000000000000000, 0.000000000000000000 ) ) ;
#12783=AXIS2_PLACEMENT_3D ( 'NONE', #11184, #4246, #8244 ) ;
#12801=CARTESIAN_POINT ( 'NONE',  ( 0.000000000000000000, 0.000000000000000000, 0.000000000000000000 ) ) ;
#12810=DIRECTION ( 'NONE',  ( 0.000000000000000000, -0.000000000000000000, 1.000000000000000000 ) ) ;
#12843=CARTESIAN_POINT ( 'NONE',  ( 1.836970198721030062E-14, 10.00000000000000000, 150.0000000000000284 ) ) ;
#12859=ADVANCED_FACE ( 'NONE', ( #4206 ), #8206, .F. ) ;
#12893=DIRECTION ( 'NONE',  ( 0.000000000000000000, 1.000000000000000000, 0.000000000000000000 ) ) ;
#12915=EDGE_LOOP ( 'NONE', ( #15328, #9212, #15567, #16555 ) ) ;
#13006=ORIENTED_EDGE ( 'NONE', *, *, #13877, .F. ) ;
#13012=ORIENTED_EDGE ( 'NONE', *, *, #15782, .T. ) ;
#13027=DIRECTION ( 'NONE',  ( 0.000000000000000000, 0.000000000000000000, 1.000000000000000000 ) ) ;
#13030=EDGE_CURVE ( 'NONE', #17219, #10404, #16273, .T. ) ;
#13055=CARTESIAN_POINT ( 'NONE',  ( 3.673940397442059178E-15, 10.00000000000000000, 30.00000000000000000 ) ) ;
#13098=ADVANCED_BREP_SHAPE_REPRESENTATION ( '', ( #15935, #8017 ), #15633 ) ;
#13105=DIRECTION ( 'NONE',  ( 0.000000000000000000, 0.000000000000000000, 1.000000000000000000 ) ) ;
#13110=DIRECTION ( 'NONE',  ( 0.000000000000000000, 0.000000000000000000, 1.000000000000000000 ) ) ;
#13114=DIRECTION ( 'NONE',  ( 0.000000000000000000, 1.000000000000000000, 0.000000000000000000 ) ) ;
#13135=LINE ( 'NONE', #7317, #74 ) ;
#13142=VERTEX_POINT ( 'NONE', #1981 ) ;
#13153=CARTESIAN_POINT ( 'NONE',  ( -36.40576474687271258, 10.00000000000000000, -26.45033635316118747 ) ) ;
#13173=ORIENTED_EDGE ( 'NONE', *, *, #8650, .F. ) ;
#13200=FACE_BOUND ( 'NONE', #17407, .T. ) ;
#13258=( NAMED_UNIT ( * ) PLANE_ANGLE_UNIT ( ) SI_UNIT ( $, .RADIAN. ) );
#13269=AXIS2_PLACEMENT_3D ( 'NONE', #3632, #9806, #6849 ) ;
#13278=AXIS2_PLACEMENT_3D ( 'NONE', #18247, #5195, #6724 ) ;
#13281=DIRECTION ( 'NONE',  ( -0.000000000000000000, 1.000000000000000000, -0.000000000000000000 ) ) ;
#13282=DIRECTION ( 'NONE',  ( -0.000000000000000000, 1.000000000000000000, -0.000000000000000000 ) ) ;
#13288=LINE ( 'NONE', #18653, #12539 ) ;
#13449=CARTESIAN_POINT ( 'NONE',  ( 0.000000000000000000, 3.000000000000000000, 0.000000000000000000 ) ) ;
#13485=PRODUCT_DEFINITION_SHAPE ( 'NONE', 'NONE',  #4673 ) ;
#13572=FACE_OUTER_BOUND ( 'NONE', #3785, .T. ) ;
#13655=DIRECTION ( 'NONE',  ( 0.000000000000000000, -0.000000000000000000, -1.000000000000000000 ) ) ;
#13664=EDGE_CURVE ( 'NONE', #15213, #7351, #5946, .T. ) ;
#13678=ADVANCED_FACE ( 'NONE', ( #11390, #14345, #15956, #13200, #18723, #9967, #2736 ), #14265, .T. ) ;
#13696=CARTESIAN_POINT ( 'NONE',  ( 13.90576474687299680, 10.00000000000000000, 42.79754323328179311 ) ) ;
#13766=UNCERTAINTY_MEASURE_WITH_UNIT (LENGTH_MEASURE( 1.000000000000000082E-05 ), #486, 'distance_accuracy_value', 'NONE');
#13812=ORIENTED_EDGE ( 'NONE', *, *, #12257, .T. ) ;
#13850=CARTESIAN_POINT ( 'NONE',  ( 0.000000000000000000, 3.000000000000000000, -150.0000000000000000 ) ) ;
#13877=EDGE_CURVE ( 'NONE', #18371, #7713, #11183, .T. ) ;
#14011=EDGE_CURVE ( 'NONE', #17219, #11928, #10522, .T. ) ;
#14018=EDGE_LOOP ( 'NONE', ( #12133, #6976 ) ) ;
#14054=VECTOR ( 'NONE', #14660, 1000.000000000000000 ) ;
#14089=ORIENTED_EDGE ( 'NONE', *, *, #17718, .T. ) ;
#14110=DIRECTION ( 'NONE',  ( -0.000000000000000000, -1.000000000000000000, -0.000000000000000000 ) ) ;
#14114=ADVANCED_FACE ( 'NONE', ( #7000, #16036, #14607, #11573, #17103, #5659, #11475 ), #2803, .F. ) ;
#14149=ORIENTED_EDGE ( 'NONE', *, *, #3310, .T. ) ;
#14173=AXIS2_PLACEMENT_3D ( 'NONE', #8531, #17475, #13110 ) ;
#14178=EDGE_LOOP ( 'NONE', ( #11967, #13012, #2605, #6713 ) ) ;
#14182=AXIS2_PLACEMENT_3D ( 'NONE', #6856, #2568, #10006 ) ;
#14191=DIRECTION ( 'NONE',  ( -0.000000000000000000, 1.000000000000000000, -0.000000000000000000 ) ) ;
#14265=PLANE ( 'NONE',  #8676 ) ;
#14280=FACE_OUTER_BOUND ( 'NONE', #10892, .T. ) ;
#14301=ORIENTED_EDGE ( 'NONE', *, *, #5157, .F. ) ;
#14324=DIRECTION ( 'NONE',  ( 0.000000000000000000, 0.000000000000000000, 1.000000000000000000 ) ) ;
#14345=FACE_BOUND ( 'NONE', #10573, .T. ) ;
#14346=DIRECTION ( 'NONE',  ( -0.000000000000000000, 1.000000000000000000, -0.000000000000000000 ) ) ;
#14360=DIRECTION ( 'NONE',  ( -0.000000000000000000, 1.000000000000000000, -0.000000000000000000 ) ) ;
#14362=VERTEX_POINT ( 'NONE', #982 ) ;
#14374=EDGE_CURVE ( 'NONE', #17109, #2107, #5365, .T. ) ;
#14393=VERTEX_POINT ( 'NONE', #15176 ) ;
#14412=SHAPE_DEFINITION_REPRESENTATION ( #13485, #16132 ) ;
#14511=AXIS2_PLACEMENT_3D ( 'NONE', #413, #2123, #13655 ) ;
#14520=ORIENTED_EDGE ( 'NONE', *, *, #14011, .F. ) ;
#14526=AXIS2_PLACEMENT_3D ( 'NONE', #17481, #15874, #70 ) ;
#14529=EDGE_CURVE ( 'NONE', #3994, #15653, #11755, .T. ) ;
#14533=ORIENTED_EDGE ( 'NONE', *, *, #17230, .T. ) ;
#14538=PRODUCT_DEFINITION_CONTEXT ( 'detailed design', #14979, 'design' ) ;
#14552=AXIS2_PLACEMENT_3D ( 'NONE', #4479, #469, #17798 ) ;
#14558=CIRCLE ( 'NONE', #9380, 2.649999999999999467 ) ;
#14577=CARTESIAN_POINT ( 'NONE',  ( 0.000000000000000000, 0.000000000000000000, 0.000000000000000000 ) ) ;
#14581=ORIENTED_EDGE ( 'NONE', *, *, #15047, .F. ) ;
#14607=FACE_BOUND ( 'NONE', #15323, .T. ) ;
#14617=CARTESIAN_POINT ( 'NONE',  ( 13.90576474687299680, 0.000000000000000000, 40.14754323328178742 ) ) ;
#14633=EDGE_LOOP ( 'NONE', ( #13006, #14760, #5121, #14089 ) ) ;
#14634=CARTESIAN_POINT ( 'NONE',  ( -36.40576474687247099, 10.00000000000000000, 26.45033635316149301 ) ) ;
#14660=DIRECTION ( 'NONE',  ( -0.000000000000000000, -1.000000000000000000, -0.000000000000000000 ) ) ;
#14760=ORIENTED_EDGE ( 'NONE', *, *, #10751, .F. ) ;
#14829=VERTEX_POINT ( 'NONE', #9780 ) ;
#14861=DIRECTION ( 'NONE',  ( -0.000000000000000000, 1.000000000000000000, -0.000000000000000000 ) ) ;
#14882=SHAPE_REPRESENTATION_RELATIONSHIP ( 'NONE' , 'NONE' ,  #16132, #13098 ) ;
#14903=ADVANCED_FACE ( 'NONE', ( #18635 ), #2253, .F. ) ;
#14943=ORIENTED_EDGE ( 'NONE', *, *, #15339, .T. ) ;
#14979=APPLICATION_CONTEXT ( 'automotive_design' ) ;
#14999=CIRCLE ( 'NONE', #6777, 55.00000000000000000 ) ;
#15028=( GEOMETRIC_REPRESENTATION_CONTEXT ( 3 ) GLOBAL_UNCERTAINTY_ASSIGNED_CONTEXT ( ( #13766 ) ) GLOBAL_UNIT_ASSIGNED_CONTEXT ( ( #486, #13258, #6396 ) ) REPRESENTATION_CONTEXT ( 'NONE', 'WORKASPACE' ) );
#15042=ORIENTED_EDGE ( 'NONE', *, *, #2891, .F. ) ;
#15047=EDGE_CURVE ( 'NONE', #16590, #18403, #18165, .T. ) ;
#15061=EDGE_CURVE ( 'NONE', #2107, #3517, #15959, .T. ) ;
#15107=FACE_OUTER_BOUND ( 'NONE', #9881, .T. ) ;
#15139=CARTESIAN_POINT ( 'NONE',  ( 13.90576474687299680, 10.00000000000000000, 42.79754323328179311 ) ) ;
#15147=AXIS2_PLACEMENT_3D ( 'NONE', #14634, #4439, #13027 ) ;
#15176=CARTESIAN_POINT ( 'NONE',  ( -36.40576474687247099, 10.00000000000000000, 23.80033635316149443 ) ) ;
#15179=FACE_OUTER_BOUND ( 'NONE', #1397, .T. ) ;
#15190=AXIS2_PLACEMENT_3D ( 'NONE', #11231, #11122, #8558 ) ;
#15200=ADVANCED_FACE ( 'NONE', ( #15107 ), #16621, .T. ) ;
#15213=VERTEX_POINT ( 'NONE', #6236 ) ;
#15228=ORIENTED_EDGE ( 'NONE', *, *, #12328, .T. ) ;
#15238=CARTESIAN_POINT ( 'NONE',  ( 45.00000000000000000, 10.00000000000000000, -5.120903701083534543E-13 ) ) ;
#15262=FACE_BOUND ( 'NONE', #7734, .T. ) ;
#15323=EDGE_LOOP ( 'NONE', ( #12491, #16910 ) ) ;
#15328=ORIENTED_EDGE ( 'NONE', *, *, #9114, .F. ) ;
#15339=EDGE_CURVE ( 'NONE', #4921, #7351, #16367, .T. ) ;
#15354=CARTESIAN_POINT ( 'NONE',  ( -36.40576474687271258, 0.000000000000000000, -29.10033635316118961 ) ) ;
#15377=VECTOR ( 'NONE', #15872, 1000.000000000000000 ) ;
#15419=ORIENTED_EDGE ( 'NONE', *, *, #15061, .F. ) ;
#15458=DIRECTION ( 'NONE',  ( 0.000000000000000000, -1.000000000000000000, 0.000000000000000000 ) ) ;
#15501=ORIENTED_EDGE ( 'NONE', *, *, #9369, .F. ) ;
#15556=DIRECTION ( 'NONE',  ( 0.000000000000000000, 1.000000000000000000, 0.000000000000000000 ) ) ;
#15567=ORIENTED_EDGE ( 'NONE', *, *, #9369, .T. ) ;
#15609=AXIS2_PLACEMENT_3D ( 'NONE', #11784, #11873, #7208 ) ;
#15633=( GEOMETRIC_REPRESENTATION_CONTEXT ( 3 ) GLOBAL_UNCERTAINTY_ASSIGNED_CONTEXT ( ( #17959 ) ) GLOBAL_UNIT_ASSIGNED_CONTEXT ( ( #11562, #4504, #10314 ) ) REPRESENTATION_CONTEXT ( 'NONE', 'WORKASPACE' ) );
#15653=VERTEX_POINT ( 'NONE', #6123 ) ;
#15679=DIRECTION ( 'NONE',  ( 0.000000000000000000, 0.000000000000000000, 1.000000000000000000 ) ) ;
#15705=CARTESIAN_POINT ( 'NONE',  ( 1.836970198721030062E-14, 10.00000000000000000, 150.0000000000000284 ) ) ;
#15736=DIRECTION ( 'NONE',  ( -0.000000000000000000, 1.000000000000000000, -0.000000000000000000 ) ) ;
#15755=DIRECTION ( 'NONE',  ( 0.000000000000000000, 0.000000000000000000, 1.000000000000000000 ) ) ;
#15759=CIRCLE ( 'NONE', #6630, 2.649999999999999467 ) ;
#15768=ADVANCED_FACE ( 'NONE', ( #15179 ), #2121, .T. ) ;
#15781=CARTESIAN_POINT ( 'NONE',  ( 45.00000000000000000, 10.00000000000000000, -2.650000000000511946 ) ) ;
#15782=EDGE_CURVE ( 'NONE', #15213, #10765, #9069, .T. ) ;
#15784=CIRCLE ( 'NONE', #7562, 2.649999999999999467 ) ;
#15787=( GEOMETRIC_REPRESENTATION_CONTEXT ( 3 ) GLOBAL_UNCERTAINTY_ASSIGNED_CONTEXT ( ( #12617 ) ) GLOBAL_UNIT_ASSIGNED_CONTEXT ( ( #4491, #4581, #16290 ) ) REPRESENTATION_CONTEXT ( 'NONE', 'WORKASPACE' ) );
#15824=CARTESIAN_POINT ( 'NONE',  ( 13.90576474687263264, 10.00000000000000000, -40.14754323328190111 ) ) ;
#15840=DIRECTION ( 'NONE',  ( 0.000000000000000000, 0.000000000000000000, 1.000000000000000000 ) ) ;
#15844=FILL_AREA_STYLE ('',( #18695 ) ) ;
#15872=DIRECTION ( 'NONE',  ( -0.000000000000000000, -1.000000000000000000, -0.000000000000000000 ) ) ;
#15874=DIRECTION ( 'NONE',  ( 0.000000000000000000, 1.000000000000000000, 0.000000000000000000 ) ) ;
#15927=CARTESIAN_POINT ( 'NONE',  ( -36.40576474687271258, 0.000000000000000000, -26.45033635316118747 ) ) ;
#15935=MANIFOLD_SOLID_BREP ( 'Cut-Extrude-Thin1', #2223 ) ;
#15956=FACE_BOUND ( 'NONE', #14018, .T. ) ;
#15959=LINE ( 'NONE', #7198, #6618 ) ;
#15968=CARTESIAN_POINT ( 'NONE',  ( 45.00000000000000000, 10.00000000000000000, -5.120903701083534543E-13 ) ) ;
#16036=FACE_BOUND ( 'NONE', #3705, .T. ) ;
#16087=DIRECTION ( 'NONE',  ( -0.000000000000000000, 1.000000000000000000, -0.000000000000000000 ) ) ;
#16107=AXIS2_PLACEMENT_3D ( 'NONE', #9867, #2534, #15679 ) ;
#16132=SHAPE_REPRESENTATION ( 'Indexing Ring', ( #8017 ), #15633 ) ;
#16152=ORIENTED_EDGE ( 'NONE', *, *, #7718, .T. ) ;
#16163=CARTESIAN_POINT ( 'NONE',  ( -36.40576474687271258, 10.00000000000000000, -23.80033635316118890 ) ) ;
#16207=CARTESIAN_POINT ( 'NONE',  ( 0.000000000000000000, 10.00000000000000000, -150.0000000000000284 ) ) ;
#16218=ADVANCED_FACE ( 'NONE', ( #5804 ), #10276, .T. ) ;
#16273=LINE ( 'NONE', #17520, #5668 ) ;
#16290=( NAMED_UNIT ( * ) SI_UNIT ( $, .STERADIAN. ) SOLID_ANGLE_UNIT ( ) );
#16367=CIRCLE ( 'NONE', #8157, 55.00000000000000000 ) ;
#16430=DIRECTION ( 'NONE',  ( -0.000000000000000000, 1.000000000000000000, -0.000000000000000000 ) ) ;
#16469=DIRECTION ( 'NONE',  ( -0.000000000000000000, 1.000000000000000000, -0.000000000000000000 ) ) ;
#16555=ORIENTED_EDGE ( 'NONE', *, *, #4185, .T. ) ;
#16590=VERTEX_POINT ( 'NONE', #8357 ) ;
#16593=CARTESIAN_POINT ( 'NONE',  ( 0.000000000000000000, 3.000000000000000000, 0.000000000000000000 ) ) ;
#16613=ORIENTED_EDGE ( 'NONE', *, *, #8434, .F. ) ;
#16621=CYLINDRICAL_SURFACE ( 'NONE', #17276, 55.00000000000000000 ) ;
#16649=ORIENTED_EDGE ( 'NONE', *, *, #14529, .T. ) ;
#16679=AXIS2_PLACEMENT_3D ( 'NONE', #12692, #14110, #18502 ) ;
#16760=ORIENTED_EDGE ( 'NONE', *, *, #18573, .T. ) ;
#16816=CIRCLE ( 'NONE', #8292, 2.649999999999999467 ) ;
#16831=EDGE_CURVE ( 'NONE', #18403, #14393, #10970, .T. ) ;
#16849=ORIENTED_EDGE ( 'NONE', *, *, #8890, .T. ) ;
#16854=DIRECTION ( 'NONE',  ( -0.000000000000000000, -1.000000000000000000, -0.000000000000000000 ) ) ;
#16876=ORIENTED_EDGE ( 'NONE', *, *, #220, .T. ) ;
#16887=DIRECTION ( 'NONE',  ( 0.000000000000000000, 0.000000000000000000, -1.000000000000000000 ) ) ;
#16890=VERTEX_POINT ( 'NONE', #6701 ) ;
#16907=ORIENTED_EDGE ( 'NONE', *, *, #9064, .T. ) ;
#16910=ORIENTED_EDGE ( 'NONE', *, *, #6119, .T. ) ;
#16947=AXIS2_PLACEMENT_3D ( 'NONE', #898, #3940, #18017 ) ;
#17030=LINE ( 'NONE', #15781, #17934 ) ;
#17103=FACE_BOUND ( 'NONE', #1029, .T. ) ;
#17106=EDGE_CURVE ( 'NONE', #11928, #17219, #4313, .T. ) ;
#17109=VERTEX_POINT ( 'NONE', #9148 ) ;
#17147=CIRCLE ( 'NONE', #12266, 2.649999999999999467 ) ;
#17154=DIRECTION ( 'NONE',  ( 0.000000000000000000, 0.000000000000000000, 1.000000000000000000 ) ) ;
#17174=CYLINDRICAL_SURFACE ( 'NONE', #17579, 2.649999999999999467 ) ;
#17196=EDGE_LOOP ( 'NONE', ( #8553, #2778, #9021, #2771 ) ) ;
#17204=CYLINDRICAL_SURFACE ( 'NONE', #14173, 2.649999999999999467 ) ;
#17206=DIRECTION ( 'NONE',  ( -0.000000000000000000, 1.000000000000000000, -0.000000000000000000 ) ) ;
#17207=EDGE_CURVE ( 'NONE', #4363, #17227, #3396, .T. ) ;
#17219=VERTEX_POINT ( 'NONE', #16207 ) ;
#17221=ORIENTED_EDGE ( 'NONE', *, *, #18549, .F. ) ;
#17226=VERTEX_POINT ( 'NONE', #7627 ) ;
#17227=VERTEX_POINT ( 'NONE', #3354 ) ;
#17230=EDGE_CURVE ( 'NONE', #10404, #9088, #2801, .T. ) ;
#17245=CARTESIAN_POINT ( 'NONE',  ( 13.90576474687299680, 10.00000000000000000, 42.79754323328179311 ) ) ;
#17276=AXIS2_PLACEMENT_3D ( 'NONE', #1765, #1859, #3585 ) ;
#17278=ORIENTED_EDGE ( 'NONE', *, *, #2891, .T. ) ;
#17375=EDGE_CURVE ( 'NONE', #8784, #10053, #13135, .T. ) ;
#17378=DIRECTION ( 'NONE',  ( 0.000000000000000000, 1.000000000000000000, 0.000000000000000000 ) ) ;
#17407=EDGE_LOOP ( 'NONE', ( #3737, #5700 ) ) ;
#17449=CARTESIAN_POINT ( 'NONE',  ( 0.000000000000000000, 10.00000000000000000, 0.000000000000000000 ) ) ;
#17475=DIRECTION ( 'NONE',  ( -0.000000000000000000, 1.000000000000000000, -0.000000000000000000 ) ) ;
#17481=CARTESIAN_POINT ( 'NONE',  ( -36.40576474687247099, 0.000000000000000000, 26.45033635316149301 ) ) ;
#17486=EDGE_CURVE ( 'NONE', #14829, #14393, #7061, .T. ) ;
#17520=CARTESIAN_POINT ( 'NONE',  ( 0.000000000000000000, 10.00000000000000000, -150.0000000000000284 ) ) ;
#17579=AXIS2_PLACEMENT_3D ( 'NONE', #5555, #2501, #11058 ) ;
#17601=EDGE_CURVE ( 'NONE', #3677, #11456, #1524, .T. ) ;
#17651=AXIS2_PLACEMENT_3D ( 'NONE', #135, #5929, #11751 ) ;
#17718=EDGE_CURVE ( 'NONE', #10053, #7713, #16816, .T. ) ;
#17798=DIRECTION ( 'NONE',  ( 0.000000000000000000, 0.000000000000000000, 1.000000000000000000 ) ) ;
#17811=CARTESIAN_POINT ( 'NONE',  ( 45.00000000000000000, 0.000000000000000000, -5.120903701083534543E-13 ) ) ;
#17837=PLANE ( 'NONE',  #14511 ) ;
#17846=DIRECTION ( 'NONE',  ( 0.000000000000000000, 0.000000000000000000, 1.000000000000000000 ) ) ;
#17854=VECTOR ( 'NONE', #14191, 1000.000000000000000 ) ;
#17870=EDGE_LOOP ( 'NONE', ( #301, #14149, #16649, #15042 ) ) ;
#17927=ADVANCED_FACE ( 'NONE', ( #14280 ), #1236, .F. ) ;
#17934=VECTOR ( 'NONE', #17206, 1000.000000000000000 ) ;
#17944=CARTESIAN_POINT ( 'NONE',  ( 13.90576474687263264, 10.00000000000000000, -42.79754323328189969 ) ) ;
#17959=UNCERTAINTY_MEASURE_WITH_UNIT (LENGTH_MEASURE( 1.000000000000000082E-05 ), #11562, 'distance_accuracy_value', 'NONE');
#17966=DIRECTION ( 'NONE',  ( -0.000000000000000000, 1.000000000000000000, -0.000000000000000000 ) ) ;
#17973=CARTESIAN_POINT ( 'NONE',  ( 45.00000000000000000, 10.00000000000000000, 2.649999999999487432 ) ) ;
#17976=ADVANCED_FACE ( 'NONE', ( #11511 ), #166, .F. ) ;
#18017=DIRECTION ( 'NONE',  ( 0.000000000000000000, 0.000000000000000000, 1.000000000000000000 ) ) ;
#18079=ORIENTED_EDGE ( 'NONE', *, *, #305, .T. ) ;
#18107=AXIS2_PLACEMENT_3D ( 'NONE', #15927, #12594, #4039 ) ;
#18151=ORIENTED_EDGE ( 'NONE', *, *, #14374, .T. ) ;
#18155=DIRECTION ( 'NONE',  ( 0.000000000000000000, 0.000000000000000000, 1.000000000000000000 ) ) ;
#18165=CIRCLE ( 'NONE', #14526, 2.649999999999999467 ) ;
#18175=EDGE_LOOP ( 'NONE', ( #5177, #4296, #18079, #15501 ) ) ;
#18247=CARTESIAN_POINT ( 'NONE',  ( 0.000000000000000000, 10.00000000000000000, 0.000000000000000000 ) ) ;
#18310=CARTESIAN_POINT ( 'NONE',  ( 0.000000000000000000, 3.000000000000000000, 0.000000000000000000 ) ) ;
#18371=VERTEX_POINT ( 'NONE', #14617 ) ;
#18403=VERTEX_POINT ( 'NONE', #5850 ) ;
#18502=DIRECTION ( 'NONE',  ( 0.000000000000000000, 0.000000000000000000, -1.000000000000000000 ) ) ;
#18515=EDGE_LOOP ( 'NONE', ( #4530, #15228, #11943, #13173 ) ) ;
#18530=CIRCLE ( 'NONE', #15190, 30.00000000000000000 ) ;
#18549=EDGE_CURVE ( 'NONE', #17226, #3517, #17147, .T. ) ;
#18559=VECTOR ( 'NONE', #8337, 1000.000000000000000 ) ;
#18573=EDGE_CURVE ( 'NONE', #17109, #17226, #1938, .T. ) ;
#18605=CARTESIAN_POINT ( 'NONE',  ( 13.90576474687299680, 10.00000000000000000, 40.14754323328178742 ) ) ;
#18635=FACE_OUTER_BOUND ( 'NONE', #1996, .T. ) ;
#18641=ORIENTED_EDGE ( 'NONE', *, *, #9468, .F. ) ;
#18643=ORIENTED_EDGE ( 'NONE', *, *, #15339, .F. ) ;
#18645=CARTESIAN_POINT ( 'NONE',  ( 13.90576474687263264, 10.00000000000000000, -42.79754323328189969 ) ) ;
#18653=CARTESIAN_POINT ( 'NONE',  ( 0.000000000000000000, 10.00000000000000000, -30.00000000000000000 ) ) ;
#18695=FILL_AREA_STYLE_COLOUR ( '', #4969 ) ;
#18720=ORIENTED_EDGE ( 'NONE', *, *, #13664, .T. ) ;
#18723=FACE_BOUND ( 'NONE', #5706, .T. ) ;
#18756=CARTESIAN_POINT ( 'NONE',  ( 0.000000000000000000, 0.000000000000000000, -55.00000000000000000 ) ) ;
#18884=COLOUR_RGB('Off White',0.89,0.88,0.83);
#18885=FILL_AREA_STYLE_COLOUR('',#18884);
#18886=FILL_AREA_STYLE('',(#18885));
#18887=SURFACE_STYLE_FILL_AREA(#18886);
#18888=SURFACE_SIDE_STYLE('',(#18887));
#18889=SURFACE_STYLE_USAGE(.BOTH.,#18888);
#18890=PRESENTATION_STYLE_ASSIGNMENT((#18889));
ENDSEC;
END-ISO-10303-21;
